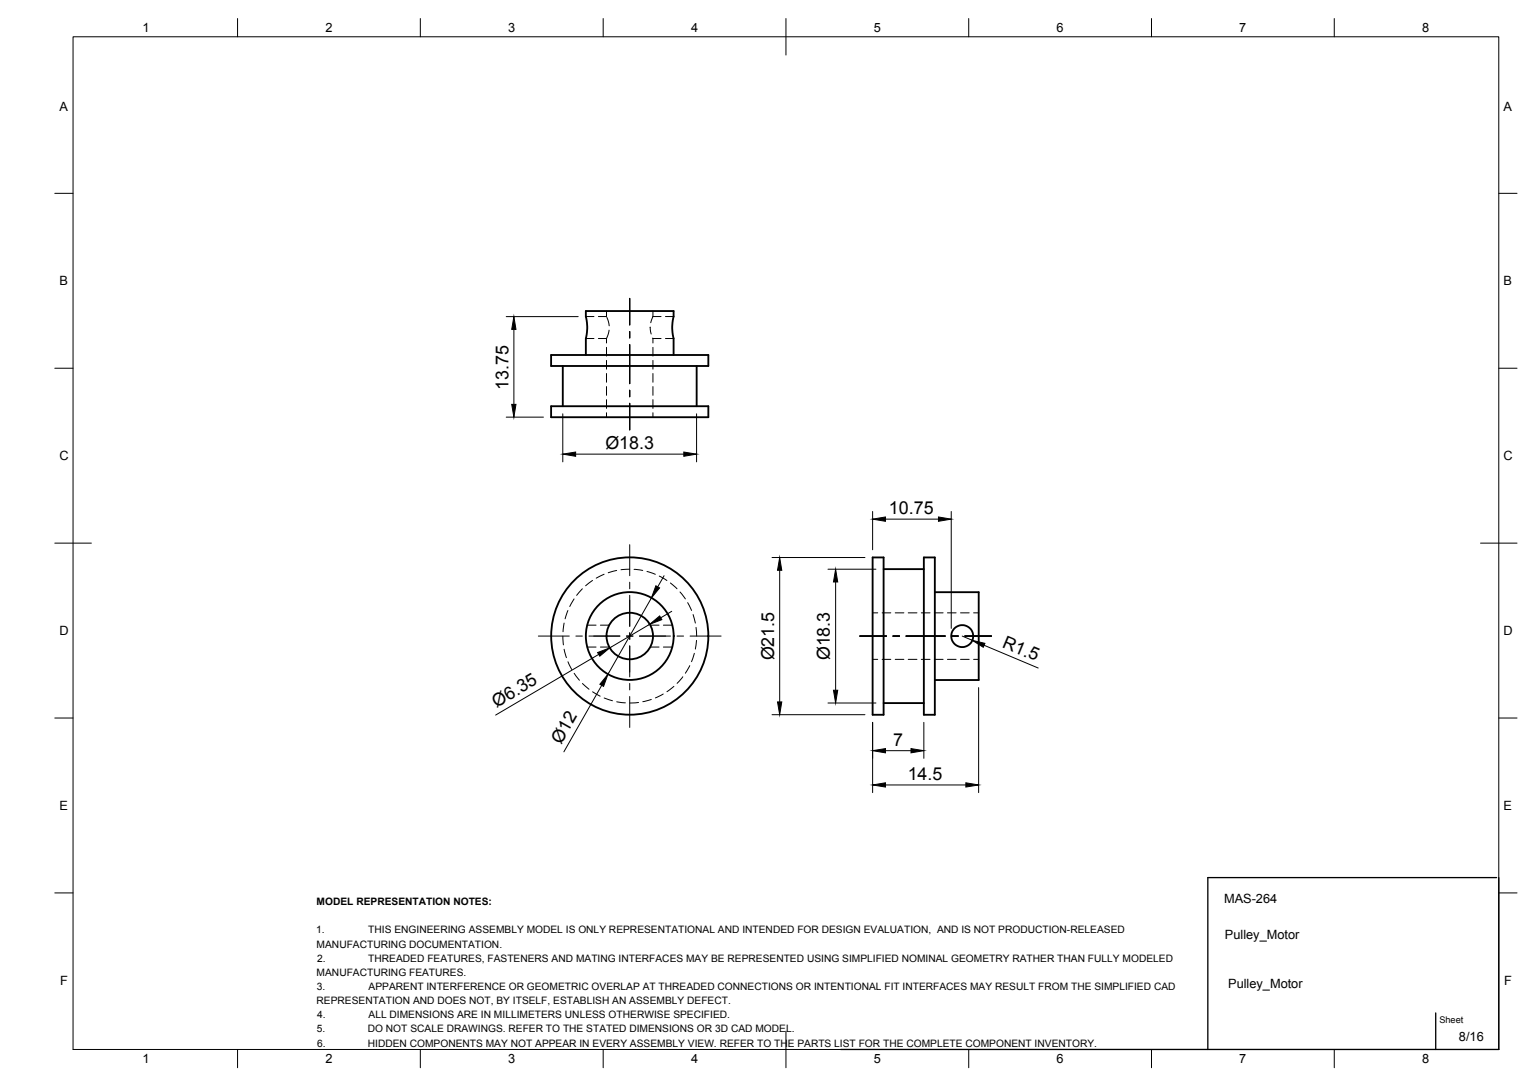
ISO-10303-21;
HEADER;
/* Generated by software containing ST-Developer
 * from STEP Tools, Inc. (www.steptools.com) 
 */

FILE_DESCRIPTION(
/* description */ (''),
/* implementation_level */ '2;1');

FILE_NAME(
/* name */ 'Pulley_Motor.step',
/* time_stamp */ '2026-10-12T15:37:13-07:00',
/* author */ (''),
/* organization */ (''),
/* preprocessor_version */ 'ST-DEVELOPER v20.2',
/* originating_system */ 'Autodesk Translation Framework v15.15.0.0',
/* authorisation */ '');

FILE_SCHEMA (('AUTOMOTIVE_DESIGN { 1 0 10303 214 3 1 1 }'));
ENDSEC;

DATA;
#10=MECHANICAL_DESIGN_GEOMETRIC_PRESENTATION_REPRESENTATION('',(#353),#36460);
#114=SHAPE_REPRESENTATION_RELATIONSHIP('SRR','None',#36526,#127);
#127=ADVANCED_BREP_SHAPE_REPRESENTATION('',(#385),#36455);
#198=FACE_BOUND('',#2211,.T.);
#199=FACE_BOUND('',#2213,.T.);
#200=FACE_BOUND('',#2215,.T.);
#201=FACE_BOUND('',#2218,.T.);
#202=FACE_BOUND('',#2221,.T.);
#203=FACE_BOUND('',#2224,.T.);
#204=FACE_BOUND('',#2226,.T.);
#353=STYLED_ITEM('',(#36598),#385);
#385=MANIFOLD_SOLID_BREP('Body1',#11289);
#660=PLANE('',#12195);
#661=PLANE('',#12197);
#662=PLANE('',#12202);
#663=PLANE('',#12210);
#664=PLANE('',#12211);
#1011=B_SPLINE_CURVE_WITH_KNOTS('',3,(#35684,#35685,#35686,#35687,#35688,
#35689,#35690,#35691,#35692,#35693,#35694,#35695,#35696,#35697,#35698,#35699,
#35700,#35701,#35702,#35703,#35704,#35705,#35706,#35707,#35708,#35709,#35710,
#35711,#35712,#35713,#35714,#35715,#35716,#35717),.UNSPECIFIED.,.T.,.F.,
(4,2,2,2,2,2,2,2,2,2,2,2,2,2,2,2,4),(0.,0.0567672348052759,0.113534469610552,
0.170293767345009,0.227053065079465,0.283812362813922,0.340571660548378,
0.397338895353654,0.45410613015893,0.510873364964206,0.567640599769482,
0.624399897503939,0.681159195238396,0.737918492972852,0.794677790707308,
0.851445025512584,0.908212260317861),.UNSPECIFIED.);
#1012=B_SPLINE_CURVE_WITH_KNOTS('',3,(#35720,#35721,#35722,#35723,#35724,
#35725,#35726,#35727,#35728,#35729,#35730,#35731,#35732,#35733,#35734,#35735,
#35736,#35737,#35738,#35739,#35740,#35741,#35742,#35743,#35744,#35745,#35746,
#35747,#35748,#35749,#35750,#35751,#35752,#35753),.UNSPECIFIED.,.T.,.F.,
(4,2,2,2,2,2,2,2,2,2,2,2,2,2,2,2,4),(-0.920290241966758,-0.862711406289492,
-0.805132570612226,-0.747675126043647,-0.690217681475069,-0.632760236906489,
-0.57530279233791,-0.517723956660645,-0.460145120983379,-0.402566285306113,
-0.344987449628848,-0.287530005060268,-0.23007256049169,-0.17261511592311,
-0.115157671354531,-0.0575788356772655,0.),.UNSPECIFIED.);
#1013=B_SPLINE_CURVE_WITH_KNOTS('',3,(#35757,#35758,#35759,#35760,#35761,
#35762,#35763,#35764,#35765,#35766),.UNSPECIFIED.,.F.,.F.,(4,2,2,2,4),(-0.230072560491689,
-0.17261511592311,-0.115157671354531,-0.0575788356772657,0.),
 .UNSPECIFIED.);
#1014=B_SPLINE_CURVE_WITH_KNOTS('',3,(#35768,#35769,#35770,#35771,#35772,
#35773,#35774,#35775,#35776,#35777,#35778,#35779,#35780,#35781,#35782,#35783,
#35784,#35785),.UNSPECIFIED.,.F.,.F.,(4,2,2,2,2,2,2,2,4),(-0.690217681475068,
-0.632760236906489,-0.57530279233791,-0.517723956660645,-0.460145120983379,
-0.402566285306113,-0.344987449628848,-0.287530005060269,-0.230072560491689),
 .UNSPECIFIED.);
#1015=B_SPLINE_CURVE_WITH_KNOTS('',3,(#35786,#35787,#35788,#35789,#35790,
#35791,#35792,#35793,#35794,#35795),.UNSPECIFIED.,.F.,.F.,(4,2,2,2,4),(0.,
0.0575788356772655,0.115157671354531,0.17261511592311,0.230072560491689),
 .UNSPECIFIED.);
#1016=B_SPLINE_CURVE_WITH_KNOTS('',3,(#35799,#35800,#35801,#35802,#35803,
#35804,#35805,#35806,#35807,#35808),.UNSPECIFIED.,.F.,.F.,(4,2,2,2,4),(0.681159195238395,
0.737918492972852,0.794677790707309,0.851445025512584,0.90821226031786),
 .UNSPECIFIED.);
#1017=B_SPLINE_CURVE_WITH_KNOTS('',3,(#35810,#35811,#35812,#35813,#35814,
#35815,#35816,#35817,#35818,#35819,#35820,#35821,#35822,#35823,#35824,#35825,
#35826,#35827),.UNSPECIFIED.,.F.,.F.,(4,2,2,2,2,2,2,2,4),(0.227053065079465,
0.283812362813922,0.340571660548378,0.397338895353654,0.45410613015893,
0.510873364964206,0.567640599769482,0.624399897503939,0.681159195238395),
 .UNSPECIFIED.);
#1018=B_SPLINE_CURVE_WITH_KNOTS('',3,(#35828,#35829,#35830,#35831,#35832,
#35833,#35834,#35835,#35836,#35837),.UNSPECIFIED.,.F.,.F.,(4,2,2,2,4),(0.90821226031786,
0.964979495123137,1.02174672992841,1.07850602766287,1.13526532539733),
 .UNSPECIFIED.);
#1528=FACE_OUTER_BOUND('',#2208,.T.);
#1529=FACE_OUTER_BOUND('',#2209,.T.);
#1530=FACE_OUTER_BOUND('',#2210,.T.);
#1531=FACE_OUTER_BOUND('',#2212,.T.);
#1532=FACE_OUTER_BOUND('',#2214,.T.);
#1533=FACE_OUTER_BOUND('',#2216,.T.);
#1534=FACE_OUTER_BOUND('',#2217,.T.);
#1535=FACE_OUTER_BOUND('',#2219,.T.);
#1536=FACE_OUTER_BOUND('',#2220,.T.);
#1537=FACE_OUTER_BOUND('',#2222,.T.);
#1538=FACE_OUTER_BOUND('',#2223,.T.);
#1539=FACE_OUTER_BOUND('',#2225,.T.);
#2208=EDGE_LOOP('',(#9836,#9837,#9838,#9839));
#2209=EDGE_LOOP('',(#9840,#9841,#9842,#9843,#9844,#9845,#9846,#9847));
#2210=EDGE_LOOP('',(#9848,#9849,#9850,#9851,#9852,#9853,#9854,#9855,#9856));
#2211=EDGE_LOOP('',(#9857));
#2212=EDGE_LOOP('',(#9858));
#2213=EDGE_LOOP('',(#9859));
#2214=EDGE_LOOP('',(#9860));
#2215=EDGE_LOOP('',(#9861));
#2216=EDGE_LOOP('',(#9862,#9863,#9864,#9865));
#2217=EDGE_LOOP('',(#9866));
#2218=EDGE_LOOP('',(#9867));
#2219=EDGE_LOOP('',(#9868,#9869,#9870,#9871));
#2220=EDGE_LOOP('',(#9872,#9873,#9874,#9875,#9876,#9877,#9878,#9879,#9880));
#2221=EDGE_LOOP('',(#9881));
#2222=EDGE_LOOP('',(#9882,#9883,#9884,#9885));
#2223=EDGE_LOOP('',(#9886));
#2224=EDGE_LOOP('',(#9887));
#2225=EDGE_LOOP('',(#9888));
#2226=EDGE_LOOP('',(#9889));
#3167=LINE('',#35719,#4113);
#3168=LINE('',#35797,#4114);
#3169=LINE('',#35841,#4115);
#3170=LINE('',#35843,#4116);
#3171=LINE('',#35856,#4117);
#3172=LINE('',#35860,#4118);
#3173=LINE('',#35865,#4119);
#3174=LINE('',#35866,#4120);
#3175=LINE('',#35871,#4121);
#4113=VECTOR('',#14722,1.5);
#4114=VECTOR('',#14725,1.5);
#4115=VECTOR('',#14730,6.00000000000002);
#4116=VECTOR('',#14731,6.00000000000002);
#4117=VECTOR('',#14748,10.75);
#4118=VECTOR('',#14753,9.15);
#4119=VECTOR('',#14760,3.17500000000003);
#4120=VECTOR('',#14761,3.17500000000003);
#4121=VECTOR('',#14766,10.75);
#4479=CIRCLE('',#12193,6.00000000000002);
#4480=CIRCLE('',#12194,6.00000000000002);
#4481=CIRCLE('',#12196,3.17500000000003);
#4482=CIRCLE('',#12198,10.75);
#4483=CIRCLE('',#12199,9.15);
#4484=CIRCLE('',#12201,10.75);
#4485=CIRCLE('',#12204,9.15);
#4486=CIRCLE('',#12206,3.17500000000003);
#4487=CIRCLE('',#12208,10.75);
#4488=CIRCLE('',#12209,10.75);
#5461=VERTEX_POINT('',#35683);
#5462=VERTEX_POINT('',#35718);
#5463=VERTEX_POINT('',#35755);
#5464=VERTEX_POINT('',#35756);
#5465=VERTEX_POINT('',#35767);
#5466=VERTEX_POINT('',#35796);
#5467=VERTEX_POINT('',#35798);
#5468=VERTEX_POINT('',#35809);
#5469=VERTEX_POINT('',#35839);
#5470=VERTEX_POINT('',#35842);
#5471=VERTEX_POINT('',#35846);
#5472=VERTEX_POINT('',#35849);
#5473=VERTEX_POINT('',#35851);
#5474=VERTEX_POINT('',#35854);
#5475=VERTEX_POINT('',#35859);
#5476=VERTEX_POINT('',#35863);
#5477=VERTEX_POINT('',#35868);
#5478=VERTEX_POINT('',#35870);
#6949=EDGE_CURVE('',#5461,#5461,#1011,.T.);
#6950=EDGE_CURVE('',#5461,#5462,#3167,.T.);
#6951=EDGE_CURVE('',#5462,#5462,#1012,.T.);
#6952=EDGE_CURVE('',#5463,#5464,#1013,.T.);
#6953=EDGE_CURVE('',#5465,#5463,#1014,.T.);
#6954=EDGE_CURVE('',#5464,#5465,#1015,.T.);
#6955=EDGE_CURVE('',#5464,#5466,#3168,.T.);
#6956=EDGE_CURVE('',#5467,#5466,#1016,.T.);
#6957=EDGE_CURVE('',#5468,#5467,#1017,.T.);
#6958=EDGE_CURVE('',#5466,#5468,#1018,.T.);
#6959=EDGE_CURVE('',#5469,#5469,#4479,.T.);
#6960=EDGE_CURVE('',#5469,#5467,#3169,.T.);
#6961=EDGE_CURVE('',#5468,#5470,#3170,.T.);
#6962=EDGE_CURVE('',#5470,#5470,#4480,.T.);
#6963=EDGE_CURVE('',#5471,#5471,#4481,.T.);
#6964=EDGE_CURVE('',#5472,#5472,#4482,.T.);
#6965=EDGE_CURVE('',#5473,#5473,#4483,.T.);
#6966=EDGE_CURVE('',#5474,#5474,#4484,.T.);
#6967=EDGE_CURVE('',#5474,#5472,#3171,.T.);
#6968=EDGE_CURVE('',#5473,#5475,#3172,.T.);
#6969=EDGE_CURVE('',#5475,#5475,#4485,.T.);
#6970=EDGE_CURVE('',#5476,#5476,#4486,.T.);
#6971=EDGE_CURVE('',#5476,#5463,#3173,.T.);
#6972=EDGE_CURVE('',#5465,#5471,#3174,.T.);
#6973=EDGE_CURVE('',#5477,#5477,#4487,.T.);
#6974=EDGE_CURVE('',#5477,#5478,#3175,.T.);
#6975=EDGE_CURVE('',#5478,#5478,#4488,.T.);
#9836=ORIENTED_EDGE('',*,*,#6949,.F.);
#9837=ORIENTED_EDGE('',*,*,#6950,.T.);
#9838=ORIENTED_EDGE('',*,*,#6951,.F.);
#9839=ORIENTED_EDGE('',*,*,#6950,.F.);
#9840=ORIENTED_EDGE('',*,*,#6952,.F.);
#9841=ORIENTED_EDGE('',*,*,#6953,.F.);
#9842=ORIENTED_EDGE('',*,*,#6954,.F.);
#9843=ORIENTED_EDGE('',*,*,#6955,.T.);
#9844=ORIENTED_EDGE('',*,*,#6956,.F.);
#9845=ORIENTED_EDGE('',*,*,#6957,.F.);
#9846=ORIENTED_EDGE('',*,*,#6958,.F.);
#9847=ORIENTED_EDGE('',*,*,#6955,.F.);
#9848=ORIENTED_EDGE('',*,*,#6959,.F.);
#9849=ORIENTED_EDGE('',*,*,#6960,.T.);
#9850=ORIENTED_EDGE('',*,*,#6956,.T.);
#9851=ORIENTED_EDGE('',*,*,#6958,.T.);
#9852=ORIENTED_EDGE('',*,*,#6961,.T.);
#9853=ORIENTED_EDGE('',*,*,#6962,.F.);
#9854=ORIENTED_EDGE('',*,*,#6961,.F.);
#9855=ORIENTED_EDGE('',*,*,#6957,.T.);
#9856=ORIENTED_EDGE('',*,*,#6960,.F.);
#9857=ORIENTED_EDGE('',*,*,#6949,.T.);
#9858=ORIENTED_EDGE('',*,*,#6959,.T.);
#9859=ORIENTED_EDGE('',*,*,#6963,.T.);
#9860=ORIENTED_EDGE('',*,*,#6964,.F.);
#9861=ORIENTED_EDGE('',*,*,#6965,.T.);
#9862=ORIENTED_EDGE('',*,*,#6966,.F.);
#9863=ORIENTED_EDGE('',*,*,#6967,.T.);
#9864=ORIENTED_EDGE('',*,*,#6964,.T.);
#9865=ORIENTED_EDGE('',*,*,#6967,.F.);
#9866=ORIENTED_EDGE('',*,*,#6966,.T.);
#9867=ORIENTED_EDGE('',*,*,#6962,.T.);
#9868=ORIENTED_EDGE('',*,*,#6965,.F.);
#9869=ORIENTED_EDGE('',*,*,#6968,.T.);
#9870=ORIENTED_EDGE('',*,*,#6969,.F.);
#9871=ORIENTED_EDGE('',*,*,#6968,.F.);
#9872=ORIENTED_EDGE('',*,*,#6970,.T.);
#9873=ORIENTED_EDGE('',*,*,#6971,.T.);
#9874=ORIENTED_EDGE('',*,*,#6952,.T.);
#9875=ORIENTED_EDGE('',*,*,#6954,.T.);
#9876=ORIENTED_EDGE('',*,*,#6972,.T.);
#9877=ORIENTED_EDGE('',*,*,#6963,.F.);
#9878=ORIENTED_EDGE('',*,*,#6972,.F.);
#9879=ORIENTED_EDGE('',*,*,#6953,.T.);
#9880=ORIENTED_EDGE('',*,*,#6971,.F.);
#9881=ORIENTED_EDGE('',*,*,#6951,.T.);
#9882=ORIENTED_EDGE('',*,*,#6973,.F.);
#9883=ORIENTED_EDGE('',*,*,#6974,.T.);
#9884=ORIENTED_EDGE('',*,*,#6975,.T.);
#9885=ORIENTED_EDGE('',*,*,#6974,.F.);
#9886=ORIENTED_EDGE('',*,*,#6973,.T.);
#9887=ORIENTED_EDGE('',*,*,#6969,.T.);
#9888=ORIENTED_EDGE('',*,*,#6975,.F.);
#9889=ORIENTED_EDGE('',*,*,#6970,.F.);
#10592=CYLINDRICAL_SURFACE('',#12190,1.5);
#10593=CYLINDRICAL_SURFACE('',#12191,1.5);
#10594=CYLINDRICAL_SURFACE('',#12192,6.00000000000002);
#10595=CYLINDRICAL_SURFACE('',#12200,10.75);
#10596=CYLINDRICAL_SURFACE('',#12203,9.15);
#10597=CYLINDRICAL_SURFACE('',#12205,3.17500000000003);
#10598=CYLINDRICAL_SURFACE('',#12207,10.75);
#11149=ADVANCED_FACE('',(#1528),#10592,.F.);
#11150=ADVANCED_FACE('',(#1529),#10593,.F.);
#11151=ADVANCED_FACE('',(#1530,#198),#10594,.T.);
#11152=ADVANCED_FACE('',(#1531,#199),#660,.T.);
#11153=ADVANCED_FACE('',(#1532,#200),#661,.F.);
#11154=ADVANCED_FACE('',(#1533),#10595,.T.);
#11155=ADVANCED_FACE('',(#1534,#201),#662,.T.);
#11156=ADVANCED_FACE('',(#1535),#10596,.T.);
#11157=ADVANCED_FACE('',(#1536,#202),#10597,.F.);
#11158=ADVANCED_FACE('',(#1537),#10598,.T.);
#11159=ADVANCED_FACE('',(#1538,#203),#663,.T.);
#11160=ADVANCED_FACE('',(#1539,#204),#664,.F.);
#11289=CLOSED_SHELL('',(#11149,#11150,#11151,#11152,#11153,#11154,#11155,
#11156,#11157,#11158,#11159,#11160));
#12189=AXIS2_PLACEMENT_3D('',#35681,#14718,#14719);
#12190=AXIS2_PLACEMENT_3D('',#35682,#14720,#14721);
#12191=AXIS2_PLACEMENT_3D('',#35754,#14723,#14724);
#12192=AXIS2_PLACEMENT_3D('',#35838,#14726,#14727);
#12193=AXIS2_PLACEMENT_3D('',#35840,#14728,#14729);
#12194=AXIS2_PLACEMENT_3D('',#35844,#14732,#14733);
#12195=AXIS2_PLACEMENT_3D('',#35845,#14734,#14735);
#12196=AXIS2_PLACEMENT_3D('',#35847,#14736,#14737);
#12197=AXIS2_PLACEMENT_3D('',#35848,#14738,#14739);
#12198=AXIS2_PLACEMENT_3D('',#35850,#14740,#14741);
#12199=AXIS2_PLACEMENT_3D('',#35852,#14742,#14743);
#12200=AXIS2_PLACEMENT_3D('',#35853,#14744,#14745);
#12201=AXIS2_PLACEMENT_3D('',#35855,#14746,#14747);
#12202=AXIS2_PLACEMENT_3D('',#35857,#14749,#14750);
#12203=AXIS2_PLACEMENT_3D('',#35858,#14751,#14752);
#12204=AXIS2_PLACEMENT_3D('',#35861,#14754,#14755);
#12205=AXIS2_PLACEMENT_3D('',#35862,#14756,#14757);
#12206=AXIS2_PLACEMENT_3D('',#35864,#14758,#14759);
#12207=AXIS2_PLACEMENT_3D('',#35867,#14762,#14763);
#12208=AXIS2_PLACEMENT_3D('',#35869,#14764,#14765);
#12209=AXIS2_PLACEMENT_3D('',#35872,#14767,#14768);
#12210=AXIS2_PLACEMENT_3D('',#35873,#14769,#14770);
#12211=AXIS2_PLACEMENT_3D('',#35874,#14771,#14772);
#14718=DIRECTION('axis',(0.,0.,1.));
#14719=DIRECTION('refdir',(1.,0.,0.));
#14720=DIRECTION('center_axis',(-1.,0.,0.));
#14721=DIRECTION('ref_axis',(0.,1.,0.));
#14722=DIRECTION('',(-1.,0.,0.));
#14723=DIRECTION('center_axis',(-1.,0.,0.));
#14724=DIRECTION('ref_axis',(0.,1.,0.));
#14725=DIRECTION('',(-1.,0.,0.));
#14726=DIRECTION('center_axis',(0.,0.,1.));
#14727=DIRECTION('ref_axis',(1.,0.,0.));
#14728=DIRECTION('center_axis',(2.24770354660149E-47,-8.64291075969854E-33,
1.));
#14729=DIRECTION('ref_axis',(1.,1.94267011675346E-79,-2.24770354660149E-47));
#14730=DIRECTION('',(0.,0.,-1.));
#14731=DIRECTION('',(0.,0.,-1.));
#14732=DIRECTION('center_axis',(1.97812547909132E-47,3.45804190325652E-32,
-1.));
#14733=DIRECTION('ref_axis',(1.,-6.84044079659716E-79,1.97812547909132E-47));
#14734=DIRECTION('center_axis',(2.24770354660149E-47,-8.64291075969854E-33,
1.));
#14735=DIRECTION('ref_axis',(1.,1.12331423616832E-95,-2.24770354660149E-47));
#14736=DIRECTION('center_axis',(-2.24770354660149E-47,8.64291075969854E-33,
-1.));
#14737=DIRECTION('ref_axis',(1.,1.94267011675346E-79,-2.24770354660149E-47));
#14738=DIRECTION('center_axis',(-1.97812547909132E-47,-3.45804190325652E-32,
1.));
#14739=DIRECTION('ref_axis',(1.,-3.6491105917259E-95,1.97812547909132E-47));
#14740=DIRECTION('center_axis',(-1.97812547909132E-47,-3.45804190325652E-32,
1.));
#14741=DIRECTION('ref_axis',(1.,-3.6491105917259E-95,1.97812547909132E-47));
#14742=DIRECTION('center_axis',(-9.86076131526267E-32,5.23079214264925E-32,
1.));
#14743=DIRECTION('ref_axis',(1.,-4.21761455916246E-79,9.86076131526267E-32));
#14744=DIRECTION('center_axis',(0.,0.,1.));
#14745=DIRECTION('ref_axis',(1.,0.,0.));
#14746=DIRECTION('center_axis',(-1.97812547909132E-47,-3.45804190325652E-32,
1.));
#14747=DIRECTION('ref_axis',(1.,-3.6491105917259E-95,1.97812547909132E-47));
#14748=DIRECTION('',(0.,0.,-1.));
#14749=DIRECTION('center_axis',(-1.97812547909132E-47,-3.45804190325652E-32,
1.));
#14750=DIRECTION('ref_axis',(1.,-3.6491105917259E-95,1.97812547909132E-47));
#14751=DIRECTION('center_axis',(0.,0.,1.));
#14752=DIRECTION('ref_axis',(1.,0.,0.));
#14753=DIRECTION('',(0.,0.,-1.));
#14754=DIRECTION('center_axis',(1.97812547909132E-47,3.45804190325652E-32,
-1.));
#14755=DIRECTION('ref_axis',(1.,-6.84044079659716E-79,1.97812547909132E-47));
#14756=DIRECTION('center_axis',(0.,0.,1.));
#14757=DIRECTION('ref_axis',(1.,0.,0.));
#14758=DIRECTION('center_axis',(-7.78296498900683E-47,-2.83123199421538E-32,
-1.));
#14759=DIRECTION('ref_axis',(1.,3.60769778730949E-95,-7.78296498900683E-47));
#14760=DIRECTION('',(0.,0.,1.));
#14761=DIRECTION('',(0.,0.,1.));
#14762=DIRECTION('center_axis',(0.,0.,1.));
#14763=DIRECTION('ref_axis',(1.,0.,0.));
#14764=DIRECTION('center_axis',(-1.97812547909132E-47,-3.45804190325652E-32,
1.));
#14765=DIRECTION('ref_axis',(1.,-3.6491105917259E-95,1.97812547909132E-47));
#14766=DIRECTION('',(0.,0.,-1.));
#14767=DIRECTION('center_axis',(-1.97812547909132E-47,-3.45804190325652E-32,
1.));
#14768=DIRECTION('ref_axis',(1.,-3.6491105917259E-95,1.97812547909132E-47));
#14769=DIRECTION('center_axis',(-1.97812547909132E-47,-3.45804190325652E-32,
1.));
#14770=DIRECTION('ref_axis',(1.,-3.6491105917259E-95,1.97812547909132E-47));
#14771=DIRECTION('center_axis',(-1.97812547909132E-47,-3.45804190325652E-32,
1.));
#14772=DIRECTION('ref_axis',(1.,-3.6491105917259E-95,1.97812547909132E-47));
#35681=CARTESIAN_POINT('',(0.,0.,0.));
#35682=CARTESIAN_POINT('Origin',(0.,-32.9435013582377,8.74200000000021));
#35683=CARTESIAN_POINT('',(-4.19052498068885,-34.4435013582377,8.74200000000021));
#35684=CARTESIAN_POINT('Ctrl Pts',(-4.19052498068884,-34.4435013582377,
8.74200000000021));
#35685=CARTESIAN_POINT('Ctrl Pts',(-4.19052498068884,-34.4435013582377,
8.9312241160178));
#35686=CARTESIAN_POINT('Ctrl Pts',(-4.1803170480147,-34.4055199393726,9.13248256201596));
#35687=CARTESIAN_POINT('Ctrl Pts',(-4.14393283331602,-34.2521973359119,
9.50179602754586));
#35688=CARTESIAN_POINT('Ctrl Pts',(-4.11833409225485,-34.1368970199764,
9.66992468182113));
#35689=CARTESIAN_POINT('Ctrl Pts',(-4.0706574299838,-33.871444598845,9.93537710295256));
#35690=CARTESIAN_POINT('Ctrl Pts',(-4.04541244329492,-33.7033082151408,
10.0506918889611));
#35691=CARTESIAN_POINT('Ctrl Pts',(-4.00984509853063,-33.3339673419624,
10.2040250565453));
#35692=CARTESIAN_POINT('Ctrl Pts',(-3.99999999999997,-33.1326990173526,
10.2420000000002));
#35693=CARTESIAN_POINT('Ctrl Pts',(-3.99999999999997,-32.7543036991228,
10.2420000000002));
#35694=CARTESIAN_POINT('Ctrl Pts',(-4.00984509853063,-32.553035374513,10.2040250565453));
#35695=CARTESIAN_POINT('Ctrl Pts',(-4.04541244329492,-32.1836945013346,
10.0506918889611));
#35696=CARTESIAN_POINT('Ctrl Pts',(-4.0706574299838,-32.0155581176304,9.93537710295256));
#35697=CARTESIAN_POINT('Ctrl Pts',(-4.11833409225485,-31.750105696499,9.66992468182113));
#35698=CARTESIAN_POINT('Ctrl Pts',(-4.14393283331602,-31.6348053805635,
9.50179602754586));
#35699=CARTESIAN_POINT('Ctrl Pts',(-4.1803170480147,-31.4814827771028,9.13248256201596));
#35700=CARTESIAN_POINT('Ctrl Pts',(-4.19052498068884,-31.4435013582377,
8.9312241160178));
#35701=CARTESIAN_POINT('Ctrl Pts',(-4.19052498068884,-31.4435013582377,
8.55277588398262));
#35702=CARTESIAN_POINT('Ctrl Pts',(-4.1803170480147,-31.4814827771028,8.35151743798446));
#35703=CARTESIAN_POINT('Ctrl Pts',(-4.14393283331602,-31.6348053805635,
7.98220397245457));
#35704=CARTESIAN_POINT('Ctrl Pts',(-4.11833409225485,-31.750105696499,7.8140753181793));
#35705=CARTESIAN_POINT('Ctrl Pts',(-4.0706574299838,-32.0155581176304,7.54862289704786));
#35706=CARTESIAN_POINT('Ctrl Pts',(-4.04541244329492,-32.1836945013346,
7.43330811103931));
#35707=CARTESIAN_POINT('Ctrl Pts',(-4.00984509853063,-32.553035374513,7.27997494345513));
#35708=CARTESIAN_POINT('Ctrl Pts',(-3.99999999999997,-32.7543036991228,
7.24200000000021));
#35709=CARTESIAN_POINT('Ctrl Pts',(-3.99999999999997,-33.1326990173526,
7.24200000000021));
#35710=CARTESIAN_POINT('Ctrl Pts',(-4.00984509853063,-33.3339673419624,
7.27997494345513));
#35711=CARTESIAN_POINT('Ctrl Pts',(-4.04541244329492,-33.7033082151408,
7.4333081110393));
#35712=CARTESIAN_POINT('Ctrl Pts',(-4.0706574299838,-33.871444598845,7.54862289704786));
#35713=CARTESIAN_POINT('Ctrl Pts',(-4.11833409225485,-34.1368970199764,
7.81407531817929));
#35714=CARTESIAN_POINT('Ctrl Pts',(-4.14393283331602,-34.2521973359119,
7.98220397245456));
#35715=CARTESIAN_POINT('Ctrl Pts',(-4.1803170480147,-34.4055199393726,8.35151743798446));
#35716=CARTESIAN_POINT('Ctrl Pts',(-4.19052498068884,-34.4435013582377,
8.55277588398262));
#35717=CARTESIAN_POINT('Ctrl Pts',(-4.19052498068884,-34.4435013582377,
8.74200000000021));
#35718=CARTESIAN_POINT('',(-7.20167460791274,-34.4435013582377,8.74200000000021));
#35719=CARTESIAN_POINT('',(0.,-34.4435013582377,8.74200000000021));
#35720=CARTESIAN_POINT('Ctrl Pts',(-7.20167460791274,-34.4435013582377,
8.74200000000021));
#35721=CARTESIAN_POINT('Ctrl Pts',(-7.20167460791274,-34.4435013582377,
8.55007054774266));
#35722=CARTESIAN_POINT('Ctrl Pts',(-7.17982819701525,-34.4045170660368,
8.34794581242564));
#35723=CARTESIAN_POINT('Ctrl Pts',(-7.10528338281718,-34.2506168512765,
7.97957260321972));
#35724=CARTESIAN_POINT('Ctrl Pts',(-7.05406308684607,-34.1358048644253,
7.81298316262817));
#35725=CARTESIAN_POINT('Ctrl Pts',(-6.96084522509015,-33.8727957338775,
7.54997403208039));
#35726=CARTESIAN_POINT('Ctrl Pts',(-6.91224663391283,-33.7061091122768,
7.43495623663964));
#35727=CARTESIAN_POINT('Ctrl Pts',(-6.84394343734937,-33.3373267297171,
7.2808923176838));
#35728=CARTESIAN_POINT('Ctrl Pts',(-6.82499999999995,-33.1350261734663,
7.24200000000021));
#35729=CARTESIAN_POINT('Ctrl Pts',(-6.82499999999995,-32.7519765430091,
7.24200000000021));
#35730=CARTESIAN_POINT('Ctrl Pts',(-6.84394343734937,-32.5496759867583,
7.28089231768381));
#35731=CARTESIAN_POINT('Ctrl Pts',(-6.91224663391283,-32.1808936041986,
7.43495623663964));
#35732=CARTESIAN_POINT('Ctrl Pts',(-6.96084522509015,-32.0142069825979,
7.54997403208039));
#35733=CARTESIAN_POINT('Ctrl Pts',(-7.05406308684607,-31.7511978520501,
7.81298316262817));
#35734=CARTESIAN_POINT('Ctrl Pts',(-7.10528338281718,-31.6363858651989,
7.97957260321973));
#35735=CARTESIAN_POINT('Ctrl Pts',(-7.17982819701525,-31.4824856504386,
8.34794581242565));
#35736=CARTESIAN_POINT('Ctrl Pts',(-7.20167460791274,-31.4435013582377,
8.55007054774266));
#35737=CARTESIAN_POINT('Ctrl Pts',(-7.20167460791274,-31.4435013582377,
8.93392945225776));
#35738=CARTESIAN_POINT('Ctrl Pts',(-7.17982819701525,-31.4824856504386,
9.13605418757478));
#35739=CARTESIAN_POINT('Ctrl Pts',(-7.10528338281718,-31.6363858651989,
9.5044273967807));
#35740=CARTESIAN_POINT('Ctrl Pts',(-7.05406308684607,-31.7511978520501,
9.67101683737225));
#35741=CARTESIAN_POINT('Ctrl Pts',(-6.96084522509015,-32.0142069825979,
9.93402596792003));
#35742=CARTESIAN_POINT('Ctrl Pts',(-6.91224663391283,-32.1808936041986,
10.0490437633608));
#35743=CARTESIAN_POINT('Ctrl Pts',(-6.84394343734937,-32.5496759867583,
10.2031076823166));
#35744=CARTESIAN_POINT('Ctrl Pts',(-6.82499999999995,-32.7519765430091,
10.2420000000002));
#35745=CARTESIAN_POINT('Ctrl Pts',(-6.82499999999995,-33.1350261734663,
10.2420000000002));
#35746=CARTESIAN_POINT('Ctrl Pts',(-6.84394343734937,-33.3373267297171,
10.2031076823166));
#35747=CARTESIAN_POINT('Ctrl Pts',(-6.91224663391283,-33.7061091122768,
10.0490437633608));
#35748=CARTESIAN_POINT('Ctrl Pts',(-6.96084522509015,-33.8727957338775,
9.93402596792003));
#35749=CARTESIAN_POINT('Ctrl Pts',(-7.05406308684607,-34.1358048644253,
9.67101683737225));
#35750=CARTESIAN_POINT('Ctrl Pts',(-7.10528338281718,-34.2506168512765,
9.50442739678069));
#35751=CARTESIAN_POINT('Ctrl Pts',(-7.17982819701525,-34.4045170660368,
9.13605418757477));
#35752=CARTESIAN_POINT('Ctrl Pts',(-7.20167460791274,-34.4435013582377,
8.93392945225776));
#35753=CARTESIAN_POINT('Ctrl Pts',(-7.20167460791274,-34.4435013582377,
8.74200000000021));
#35754=CARTESIAN_POINT('Origin',(0.,-32.9435013582377,8.74200000000021));
#35755=CARTESIAN_POINT('',(-13.175,-32.9435013582377,7.24200000000021));
#35756=CARTESIAN_POINT('',(-12.7983253920872,-34.4435013582377,8.74200000000021));
#35757=CARTESIAN_POINT('Ctrl Pts',(-13.175,-32.9435013582377,7.24200000000021));
#35758=CARTESIAN_POINT('Ctrl Pts',(-13.175,-33.1350261734663,7.24200000000021));
#35759=CARTESIAN_POINT('Ctrl Pts',(-13.1560565626506,-33.3373267297171,
7.2808923176838));
#35760=CARTESIAN_POINT('Ctrl Pts',(-13.0877533660871,-33.7061091122768,
7.43495623663964));
#35761=CARTESIAN_POINT('Ctrl Pts',(-13.0391547749098,-33.8727957338775,
7.54997403208039));
#35762=CARTESIAN_POINT('Ctrl Pts',(-12.9459369131539,-34.1358048644253,
7.81298316262817));
#35763=CARTESIAN_POINT('Ctrl Pts',(-12.8947166171828,-34.2506168512765,
7.97957260321972));
#35764=CARTESIAN_POINT('Ctrl Pts',(-12.8201718029847,-34.4045170660368,
8.34794581242564));
#35765=CARTESIAN_POINT('Ctrl Pts',(-12.7983253920872,-34.4435013582377,
8.55007054774266));
#35766=CARTESIAN_POINT('Ctrl Pts',(-12.7983253920872,-34.4435013582377,
8.74200000000021));
#35767=CARTESIAN_POINT('',(-13.175,-32.9435013582377,10.2420000000002));
#35768=CARTESIAN_POINT('Ctrl Pts',(-13.175,-32.9435013582377,10.2420000000002));
#35769=CARTESIAN_POINT('Ctrl Pts',(-13.175,-32.7519765430091,10.2420000000002));
#35770=CARTESIAN_POINT('Ctrl Pts',(-13.1560565626506,-32.5496759867583,
10.2031076823166));
#35771=CARTESIAN_POINT('Ctrl Pts',(-13.0877533660871,-32.1808936041986,
10.0490437633608));
#35772=CARTESIAN_POINT('Ctrl Pts',(-13.0391547749098,-32.0142069825979,
9.93402596792003));
#35773=CARTESIAN_POINT('Ctrl Pts',(-12.9459369131539,-31.7511978520501,
9.67101683737225));
#35774=CARTESIAN_POINT('Ctrl Pts',(-12.8947166171828,-31.6363858651989,
9.5044273967807));
#35775=CARTESIAN_POINT('Ctrl Pts',(-12.8201718029847,-31.4824856504386,
9.13605418757478));
#35776=CARTESIAN_POINT('Ctrl Pts',(-12.7983253920872,-31.4435013582377,
8.93392945225776));
#35777=CARTESIAN_POINT('Ctrl Pts',(-12.7983253920872,-31.4435013582377,
8.55007054774266));
#35778=CARTESIAN_POINT('Ctrl Pts',(-12.8201718029847,-31.4824856504386,
8.34794581242564));
#35779=CARTESIAN_POINT('Ctrl Pts',(-12.8947166171828,-31.6363858651989,
7.97957260321972));
#35780=CARTESIAN_POINT('Ctrl Pts',(-12.9459369131539,-31.7511978520501,
7.81298316262817));
#35781=CARTESIAN_POINT('Ctrl Pts',(-13.0391547749098,-32.0142069825979,
7.54997403208039));
#35782=CARTESIAN_POINT('Ctrl Pts',(-13.0877533660871,-32.1808936041986,
7.43495623663964));
#35783=CARTESIAN_POINT('Ctrl Pts',(-13.1560565626506,-32.5496759867583,
7.28089231768381));
#35784=CARTESIAN_POINT('Ctrl Pts',(-13.175,-32.7519765430091,7.24200000000021));
#35785=CARTESIAN_POINT('Ctrl Pts',(-13.175,-32.9435013582377,7.24200000000021));
#35786=CARTESIAN_POINT('Ctrl Pts',(-12.7983253920872,-34.4435013582377,
8.74200000000021));
#35787=CARTESIAN_POINT('Ctrl Pts',(-12.7983253920872,-34.4435013582377,
8.93392945225776));
#35788=CARTESIAN_POINT('Ctrl Pts',(-12.8201718029847,-34.4045170660368,
9.13605418757477));
#35789=CARTESIAN_POINT('Ctrl Pts',(-12.8947166171828,-34.2506168512765,
9.5044273967807));
#35790=CARTESIAN_POINT('Ctrl Pts',(-12.9459369131539,-34.1358048644253,
9.67101683737225));
#35791=CARTESIAN_POINT('Ctrl Pts',(-13.0391547749098,-33.8727957338775,
9.93402596792003));
#35792=CARTESIAN_POINT('Ctrl Pts',(-13.0877533660871,-33.7061091122768,
10.0490437633608));
#35793=CARTESIAN_POINT('Ctrl Pts',(-13.1560565626506,-33.3373267297171,
10.2031076823166));
#35794=CARTESIAN_POINT('Ctrl Pts',(-13.175,-33.1350261734663,10.2420000000002));
#35795=CARTESIAN_POINT('Ctrl Pts',(-13.175,-32.9435013582377,10.2420000000002));
#35796=CARTESIAN_POINT('',(-15.8094750193111,-34.4435013582377,8.74200000000021));
#35797=CARTESIAN_POINT('',(0.,-34.4435013582377,8.74200000000021));
#35798=CARTESIAN_POINT('',(-16.,-32.9435013582377,10.2420000000002));
#35799=CARTESIAN_POINT('Ctrl Pts',(-16.,-32.9435013582377,10.2420000000002));
#35800=CARTESIAN_POINT('Ctrl Pts',(-16.,-33.1326990173526,10.2420000000002));
#35801=CARTESIAN_POINT('Ctrl Pts',(-15.9901549014694,-33.3339673419624,
10.2040250565453));
#35802=CARTESIAN_POINT('Ctrl Pts',(-15.9545875567051,-33.7033082151408,
10.0506918889611));
#35803=CARTESIAN_POINT('Ctrl Pts',(-15.9293425700162,-33.871444598845,9.93537710295256));
#35804=CARTESIAN_POINT('Ctrl Pts',(-15.8816659077451,-34.1368970199764,
9.66992468182113));
#35805=CARTESIAN_POINT('Ctrl Pts',(-15.856067166684,-34.2521973359119,9.50179602754586));
#35806=CARTESIAN_POINT('Ctrl Pts',(-15.8196829519853,-34.4055199393726,
9.13248256201596));
#35807=CARTESIAN_POINT('Ctrl Pts',(-15.8094750193111,-34.4435013582377,
8.9312241160178));
#35808=CARTESIAN_POINT('Ctrl Pts',(-15.8094750193111,-34.4435013582377,
8.74200000000021));
#35809=CARTESIAN_POINT('',(-16.,-32.9435013582377,7.24200000000021));
#35810=CARTESIAN_POINT('Ctrl Pts',(-16.,-32.9435013582377,7.24200000000021));
#35811=CARTESIAN_POINT('Ctrl Pts',(-16.,-32.7543036991228,7.24200000000021));
#35812=CARTESIAN_POINT('Ctrl Pts',(-15.9901549014694,-32.553035374513,7.27997494345513));
#35813=CARTESIAN_POINT('Ctrl Pts',(-15.9545875567051,-32.1836945013346,
7.43330811103931));
#35814=CARTESIAN_POINT('Ctrl Pts',(-15.9293425700162,-32.0155581176304,
7.54862289704786));
#35815=CARTESIAN_POINT('Ctrl Pts',(-15.8816659077451,-31.750105696499,7.8140753181793));
#35816=CARTESIAN_POINT('Ctrl Pts',(-15.856067166684,-31.6348053805635,7.98220397245456));
#35817=CARTESIAN_POINT('Ctrl Pts',(-15.8196829519853,-31.4814827771028,
8.35151743798446));
#35818=CARTESIAN_POINT('Ctrl Pts',(-15.8094750193111,-31.4435013582377,
8.55277588398262));
#35819=CARTESIAN_POINT('Ctrl Pts',(-15.8094750193111,-31.4435013582377,
8.9312241160178));
#35820=CARTESIAN_POINT('Ctrl Pts',(-15.8196829519853,-31.4814827771028,
9.13248256201596));
#35821=CARTESIAN_POINT('Ctrl Pts',(-15.856067166684,-31.6348053805635,9.50179602754586));
#35822=CARTESIAN_POINT('Ctrl Pts',(-15.8816659077451,-31.750105696499,9.66992468182113));
#35823=CARTESIAN_POINT('Ctrl Pts',(-15.9293425700162,-32.0155581176304,
9.93537710295256));
#35824=CARTESIAN_POINT('Ctrl Pts',(-15.9545875567051,-32.1836945013346,
10.0506918889611));
#35825=CARTESIAN_POINT('Ctrl Pts',(-15.9901549014694,-32.553035374513,10.2040250565453));
#35826=CARTESIAN_POINT('Ctrl Pts',(-16.,-32.7543036991228,10.2420000000002));
#35827=CARTESIAN_POINT('Ctrl Pts',(-16.,-32.9435013582377,10.2420000000002));
#35828=CARTESIAN_POINT('Ctrl Pts',(-15.8094750193111,-34.4435013582377,
8.74200000000021));
#35829=CARTESIAN_POINT('Ctrl Pts',(-15.8094750193111,-34.4435013582377,
8.55277588398262));
#35830=CARTESIAN_POINT('Ctrl Pts',(-15.8196829519853,-34.4055199393726,
8.35151743798446));
#35831=CARTESIAN_POINT('Ctrl Pts',(-15.856067166684,-34.2521973359119,7.98220397245456));
#35832=CARTESIAN_POINT('Ctrl Pts',(-15.8816659077451,-34.1368970199764,
7.81407531817929));
#35833=CARTESIAN_POINT('Ctrl Pts',(-15.9293425700162,-33.871444598845,7.54862289704786));
#35834=CARTESIAN_POINT('Ctrl Pts',(-15.9545875567051,-33.7033082151408,
7.4333081110393));
#35835=CARTESIAN_POINT('Ctrl Pts',(-15.9901549014694,-33.3339673419624,
7.27997494345513));
#35836=CARTESIAN_POINT('Ctrl Pts',(-16.,-33.1326990173526,7.24200000000021));
#35837=CARTESIAN_POINT('Ctrl Pts',(-16.,-32.9435013582377,7.24200000000021));
#35838=CARTESIAN_POINT('Origin',(-9.99999999999999,-32.9435013582377,-3.50799999999979));
#35839=CARTESIAN_POINT('',(-16.,-32.9435013582377,10.9920000000002));
#35840=CARTESIAN_POINT('Origin',(-9.99999999999999,-32.9435013582377,10.9920000000002));
#35841=CARTESIAN_POINT('',(-16.,-32.9435013582377,-3.50799999999979));
#35842=CARTESIAN_POINT('',(-16.,-32.9435013582377,4.99200000000021));
#35843=CARTESIAN_POINT('',(-16.,-32.9435013582377,-3.50799999999979));
#35844=CARTESIAN_POINT('Origin',(-9.99999999999999,-32.9435013582377,4.99200000000021));
#35845=CARTESIAN_POINT('Origin',(-10.,-32.9435013582377,10.9920000000002));
#35846=CARTESIAN_POINT('',(-13.175,-32.9435013582377,10.9920000000002));
#35847=CARTESIAN_POINT('Origin',(-9.99999999999998,-32.9435013582377,10.9920000000002));
#35848=CARTESIAN_POINT('Origin',(-10.,-32.9435013582377,3.49200000000021));
#35849=CARTESIAN_POINT('',(-20.75,-32.9435013582377,3.49200000000021));
#35850=CARTESIAN_POINT('Origin',(-10.,-32.9435013582377,3.49200000000021));
#35851=CARTESIAN_POINT('',(-19.15,-32.9435013582377,3.49200000000021));
#35852=CARTESIAN_POINT('Origin',(-9.99999999999996,-32.9435013582377,3.49200000000021));
#35853=CARTESIAN_POINT('Origin',(-10.,-32.9435013582377,3.49200000000021));
#35854=CARTESIAN_POINT('',(-20.75,-32.9435013582377,4.99200000000021));
#35855=CARTESIAN_POINT('Origin',(-10.,-32.9435013582377,4.99200000000021));
#35856=CARTESIAN_POINT('',(-20.75,-32.9435013582377,3.49200000000021));
#35857=CARTESIAN_POINT('Origin',(-10.,-32.9435013582377,4.99200000000021));
#35858=CARTESIAN_POINT('Origin',(-9.99999999999996,-32.9435013582377,-3.50799999999979));
#35859=CARTESIAN_POINT('',(-19.15,-32.9435013582377,-2.00799999999979));
#35860=CARTESIAN_POINT('',(-19.15,-32.9435013582377,-3.50799999999979));
#35861=CARTESIAN_POINT('Origin',(-9.99999999999996,-32.9435013582377,-2.00799999999979));
#35862=CARTESIAN_POINT('Origin',(-9.99999999999998,-32.9435013582377,-3.50799999999979));
#35863=CARTESIAN_POINT('',(-13.175,-32.9435013582377,-3.50799999999979));
#35864=CARTESIAN_POINT('Origin',(-9.99999999999998,-32.9435013582377,-3.50799999999979));
#35865=CARTESIAN_POINT('',(-13.175,-32.9435013582377,-3.50799999999979));
#35866=CARTESIAN_POINT('',(-13.175,-32.9435013582377,-3.50799999999979));
#35867=CARTESIAN_POINT('Origin',(-10.,-32.9435013582377,-3.50799999999979));
#35868=CARTESIAN_POINT('',(-20.75,-32.9435013582377,-2.00799999999979));
#35869=CARTESIAN_POINT('Origin',(-10.,-32.9435013582377,-2.00799999999979));
#35870=CARTESIAN_POINT('',(-20.75,-32.9435013582377,-3.50799999999979));
#35871=CARTESIAN_POINT('',(-20.75,-32.9435013582377,-3.50799999999979));
#35872=CARTESIAN_POINT('Origin',(-10.,-32.9435013582377,-3.50799999999979));
#35873=CARTESIAN_POINT('Origin',(-10.,-32.9435013582377,-2.00799999999979));
#35874=CARTESIAN_POINT('Origin',(-10.,-32.9435013582377,-3.50799999999979));
#36439=UNCERTAINTY_MEASURE_WITH_UNIT(LENGTH_MEASURE(0.01),#36461,
'DISTANCE_ACCURACY_VALUE',
'Maximum model space distance between geometric entities at asserted c
onnectivities');
#36444=UNCERTAINTY_MEASURE_WITH_UNIT(LENGTH_MEASURE(0.01),#36461,
'DISTANCE_ACCURACY_VALUE',
'Maximum model space distance between geometric entities at asserted c
onnectivities');
#36455=(
GEOMETRIC_REPRESENTATION_CONTEXT(3)
GLOBAL_UNCERTAINTY_ASSIGNED_CONTEXT((#36439))
GLOBAL_UNIT_ASSIGNED_CONTEXT((#36461,#36463,#36464))
REPRESENTATION_CONTEXT('','3D')
);
#36460=(
GEOMETRIC_REPRESENTATION_CONTEXT(3)
GLOBAL_UNCERTAINTY_ASSIGNED_CONTEXT((#36444))
GLOBAL_UNIT_ASSIGNED_CONTEXT((#36461,#36463,#36464))
REPRESENTATION_CONTEXT('','3D')
);
#36461=(
LENGTH_UNIT()
NAMED_UNIT(*)
SI_UNIT(.MILLI.,.METRE.)
);
#36463=(
NAMED_UNIT(*)
PLANE_ANGLE_UNIT()
SI_UNIT($,.RADIAN.)
);
#36464=(
NAMED_UNIT(*)
SI_UNIT($,.STERADIAN.)
SOLID_ANGLE_UNIT()
);
#36475=SHAPE_DEFINITION_REPRESENTATION(#36495,#36526);
#36495=PRODUCT_DEFINITION_SHAPE('',$,#36542);
#36526=SHAPE_REPRESENTATION('',(#12189),#36455);
#36531=PRODUCT_DEFINITION_CONTEXT('part definition',#36578,'design');
#36542=PRODUCT_DEFINITION('Pulley_Motor','Pulley_Motor',#36557,#36531);
#36557=PRODUCT_DEFINITION_FORMATION('',$,#36590);
#36578=APPLICATION_CONTEXT(
'Core Data for Automotive Mechanical Design Process');
#36579=PRODUCT_CONTEXT('part definition',#36578,'mechanical');
#36590=PRODUCT('Pulley_Motor','Pulley_Motor',$,(#36579));
#36598=PRESENTATION_STYLE_ASSIGNMENT((#36603));
#36603=SURFACE_STYLE_USAGE(.BOTH.,#36608);
#36608=SURFACE_SIDE_STYLE('',(#36613));
#36613=SURFACE_STYLE_FILL_AREA(#36618);
#36618=FILL_AREA_STYLE('Opaque(245,245,246)',(#36623));
#36623=FILL_AREA_STYLE_COLOUR('Opaque(245,245,246)',#36628);
#36628=COLOUR_RGB('Opaque(245,245,246)', 0.40784314, 0.44705882, 0.49803922);
ENDSEC;
END-ISO-10303-21;
